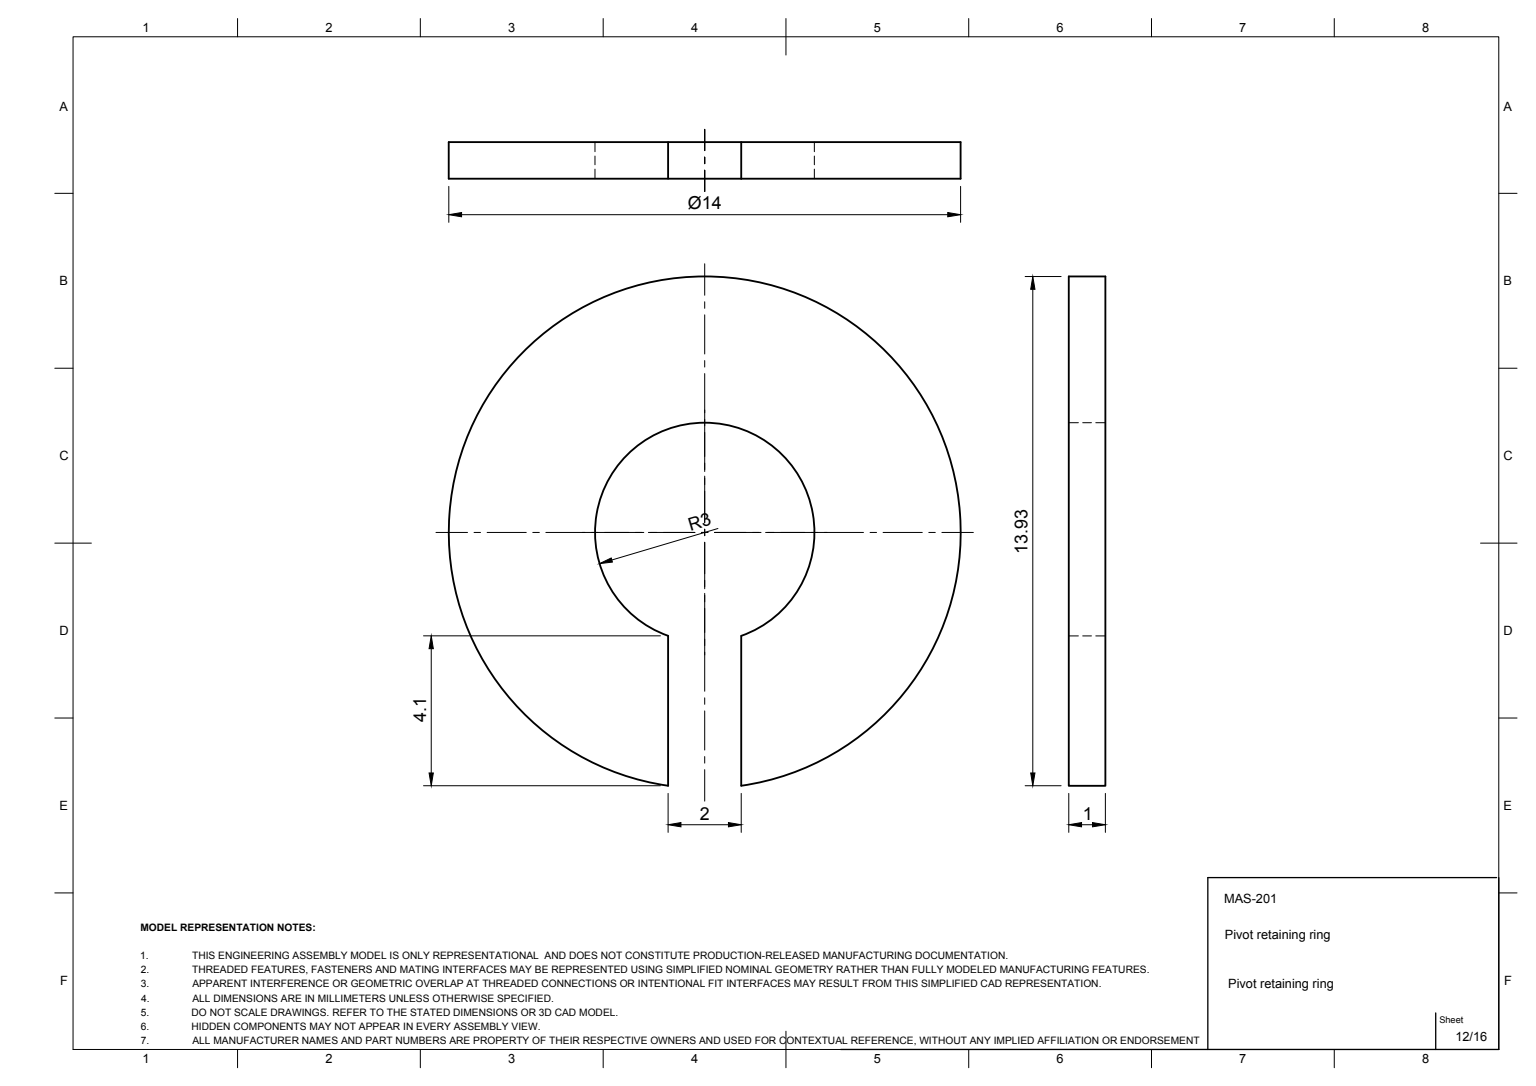
ISO-10303-21;
HEADER;
/* Generated by software containing ST-Developer
 * from STEP Tools, Inc. (www.steptools.com) 
 */

FILE_DESCRIPTION(
/* description */ ('Independent manual two-gate roller-track escapement for nominal30mm d
iameter20mm wide feed rollers. Opposed gates are driven by native capt
ured pin-slot loops with positive curved-slot travel stops at\X\B116de
g. Repeated gate/pin/washer/clip instances, adapted native common bear
ing families, full retaining lips and rotating polymer grip. External 
workpieces, gravity feeder/incline and mount anchors outside assembly.
 No powered-feed compatibility, impact, capacity, safety, force, wear 
or life rating.'),
/* implementation_level */ '2;1');

FILE_NAME(
/* name */ 'Pivot retaining ring.step',
/* time_stamp */ '2026-11-08T18:43:23-08:00',
/* author */ (''),
/* organization */ (''),
/* preprocessor_version */ 'ST-DEVELOPER v20.2',
/* originating_system */ 'Autodesk Translation Framework v15.17.0.0',
/* authorisation */ '');

FILE_SCHEMA (('AUTOMOTIVE_DESIGN { 1 0 10303 214 3 1 1 }'));
ENDSEC;

DATA;
#10=MECHANICAL_DESIGN_GEOMETRIC_PRESENTATION_REPRESENTATION('',(#466),#19863);
#428=SHAPE_REPRESENTATION_RELATIONSHIP('SRR','None',#19946,#447);
#447=ADVANCED_BREP_SHAPE_REPRESENTATION('',(#485),#19855);
#466=STYLED_ITEM('',(#20044),#485);
#485=MANIFOLD_SOLID_BREP('Body1',#6435);
#850=LINE('',#15919,#1315);
#851=LINE('',#15921,#1316);
#852=LINE('',#15923,#1317);
#853=LINE('',#15924,#1318);
#854=LINE('',#15928,#1319);
#855=LINE('',#15930,#1320);
#856=LINE('',#15932,#1321);
#857=LINE('',#15933,#1322);
#1315=VECTOR('',#8264,10.);
#1316=VECTOR('',#8265,10.);
#1317=VECTOR('',#8266,10.);
#1318=VECTOR('',#8267,10.);
#1319=VECTOR('',#8270,10.);
#1320=VECTOR('',#8271,10.);
#1321=VECTOR('',#8272,10.);
#1322=VECTOR('',#8273,10.);
#1554=CYLINDRICAL_SURFACE('',#7015,3.);
#1555=CYLINDRICAL_SURFACE('',#7017,7.);
#1937=FACE_OUTER_BOUND('',#2352,.T.);
#1938=FACE_OUTER_BOUND('',#2353,.T.);
#1939=FACE_OUTER_BOUND('',#2354,.T.);
#1940=FACE_OUTER_BOUND('',#2355,.T.);
#1941=FACE_OUTER_BOUND('',#2356,.T.);
#1942=FACE_OUTER_BOUND('',#2357,.T.);
#2352=EDGE_LOOP('',(#5409,#5410,#5411,#5412));
#2353=EDGE_LOOP('',(#5413,#5414,#5415,#5416));
#2354=EDGE_LOOP('',(#5417,#5418,#5419,#5420));
#2355=EDGE_LOOP('',(#5421,#5422,#5423,#5424));
#2356=EDGE_LOOP('',(#5425,#5426,#5427,#5428));
#2357=EDGE_LOOP('',(#5429,#5430,#5431,#5432));
#2574=CIRCLE('',#7013,7.);
#2575=CIRCLE('',#7014,3.);
#2576=CIRCLE('',#7016,3.);
#2577=CIRCLE('',#7018,7.);
#3048=VERTEX_POINT('',#15917);
#3049=VERTEX_POINT('',#15918);
#3050=VERTEX_POINT('',#15920);
#3051=VERTEX_POINT('',#15922);
#3052=VERTEX_POINT('',#15926);
#3053=VERTEX_POINT('',#15927);
#3054=VERTEX_POINT('',#15929);
#3055=VERTEX_POINT('',#15931);
#3863=EDGE_CURVE('',#3048,#3049,#850,.T.);
#3864=EDGE_CURVE('',#3050,#3048,#851,.T.);
#3865=EDGE_CURVE('',#3051,#3050,#852,.T.);
#3866=EDGE_CURVE('',#3049,#3051,#853,.T.);
#3867=EDGE_CURVE('',#3052,#3053,#854,.T.);
#3868=EDGE_CURVE('',#3054,#3052,#855,.T.);
#3869=EDGE_CURVE('',#3055,#3054,#856,.T.);
#3870=EDGE_CURVE('',#3053,#3055,#857,.T.);
#3871=EDGE_CURVE('',#3050,#3055,#2574,.T.);
#3872=EDGE_CURVE('',#3053,#3048,#2575,.T.);
#3873=EDGE_CURVE('',#3052,#3049,#2576,.T.);
#3874=EDGE_CURVE('',#3051,#3054,#2577,.T.);
#5409=ORIENTED_EDGE('',*,*,#3863,.F.);
#5410=ORIENTED_EDGE('',*,*,#3864,.F.);
#5411=ORIENTED_EDGE('',*,*,#3865,.F.);
#5412=ORIENTED_EDGE('',*,*,#3866,.F.);
#5413=ORIENTED_EDGE('',*,*,#3867,.F.);
#5414=ORIENTED_EDGE('',*,*,#3868,.F.);
#5415=ORIENTED_EDGE('',*,*,#3869,.F.);
#5416=ORIENTED_EDGE('',*,*,#3870,.F.);
#5417=ORIENTED_EDGE('',*,*,#3870,.T.);
#5418=ORIENTED_EDGE('',*,*,#3871,.F.);
#5419=ORIENTED_EDGE('',*,*,#3864,.T.);
#5420=ORIENTED_EDGE('',*,*,#3872,.F.);
#5421=ORIENTED_EDGE('',*,*,#3867,.T.);
#5422=ORIENTED_EDGE('',*,*,#3872,.T.);
#5423=ORIENTED_EDGE('',*,*,#3863,.T.);
#5424=ORIENTED_EDGE('',*,*,#3873,.F.);
#5425=ORIENTED_EDGE('',*,*,#3869,.T.);
#5426=ORIENTED_EDGE('',*,*,#3874,.F.);
#5427=ORIENTED_EDGE('',*,*,#3865,.T.);
#5428=ORIENTED_EDGE('',*,*,#3871,.T.);
#5429=ORIENTED_EDGE('',*,*,#3868,.T.);
#5430=ORIENTED_EDGE('',*,*,#3873,.T.);
#5431=ORIENTED_EDGE('',*,*,#3866,.T.);
#5432=ORIENTED_EDGE('',*,*,#3874,.T.);
#6026=PLANE('',#7010);
#6027=PLANE('',#7011);
#6028=PLANE('',#7012);
#6029=PLANE('',#7019);
#6316=ADVANCED_FACE('',(#1937),#6026,.F.);
#6317=ADVANCED_FACE('',(#1938),#6027,.F.);
#6318=ADVANCED_FACE('',(#1939),#6028,.F.);
#6319=ADVANCED_FACE('',(#1940),#1554,.F.);
#6320=ADVANCED_FACE('',(#1941),#1555,.T.);
#6321=ADVANCED_FACE('',(#1942),#6029,.T.);
#6435=CLOSED_SHELL('',(#6316,#6317,#6318,#6319,#6320,#6321));
#7009=AXIS2_PLACEMENT_3D('',#15915,#8260,#8261);
#7010=AXIS2_PLACEMENT_3D('',#15916,#8262,#8263);
#7011=AXIS2_PLACEMENT_3D('',#15925,#8268,#8269);
#7012=AXIS2_PLACEMENT_3D('',#15934,#8274,#8275);
#7013=AXIS2_PLACEMENT_3D('',#15935,#8276,#8277);
#7014=AXIS2_PLACEMENT_3D('',#15936,#8278,#8279);
#7015=AXIS2_PLACEMENT_3D('',#15937,#8280,#8281);
#7016=AXIS2_PLACEMENT_3D('',#15938,#8282,#8283);
#7017=AXIS2_PLACEMENT_3D('',#15939,#8284,#8285);
#7018=AXIS2_PLACEMENT_3D('',#15940,#8286,#8287);
#7019=AXIS2_PLACEMENT_3D('',#15941,#8288,#8289);
#8260=DIRECTION('axis',(0.,0.,1.));
#8261=DIRECTION('refdir',(1.,0.,0.));
#8262=DIRECTION('center_axis',(-1.,0.,0.));
#8263=DIRECTION('ref_axis',(0.,1.,0.));
#8264=DIRECTION('',(0.,0.,1.));
#8265=DIRECTION('',(0.,-1.,0.));
#8266=DIRECTION('',(0.,0.,-1.));
#8267=DIRECTION('',(0.,1.,0.));
#8268=DIRECTION('center_axis',(1.,0.,0.));
#8269=DIRECTION('ref_axis',(0.,-1.,0.));
#8270=DIRECTION('',(0.,0.,-1.));
#8271=DIRECTION('',(0.,-1.,0.));
#8272=DIRECTION('',(0.,0.,1.));
#8273=DIRECTION('',(0.,1.,0.));
#8274=DIRECTION('center_axis',(0.,0.,1.));
#8275=DIRECTION('ref_axis',(1.,0.,0.));
#8276=DIRECTION('center_axis',(0.,0.,1.));
#8277=DIRECTION('ref_axis',(1.,0.,0.));
#8278=DIRECTION('center_axis',(0.,0.,-1.));
#8279=DIRECTION('ref_axis',(1.,0.,0.));
#8280=DIRECTION('center_axis',(0.,0.,1.));
#8281=DIRECTION('ref_axis',(6.12323399573677E-17,-1.,0.));
#8282=DIRECTION('center_axis',(0.,0.,-1.));
#8283=DIRECTION('ref_axis',(1.,0.,0.));
#8284=DIRECTION('center_axis',(0.,0.,1.));
#8285=DIRECTION('ref_axis',(6.12323399573677E-17,-1.,0.));
#8286=DIRECTION('center_axis',(0.,0.,1.));
#8287=DIRECTION('ref_axis',(1.,0.,0.));
#8288=DIRECTION('center_axis',(0.,0.,1.));
#8289=DIRECTION('ref_axis',(1.,0.,0.));
#15915=CARTESIAN_POINT('',(0.,0.,0.));
#15916=CARTESIAN_POINT('Origin',(-1.,0.,1.));
#15917=CARTESIAN_POINT('',(-1.,2.82842712474619,0.));
#15918=CARTESIAN_POINT('',(-1.,2.82842712474619,1.));
#15919=CARTESIAN_POINT('',(-1.,2.82842712474619,0.));
#15920=CARTESIAN_POINT('',(-1.,6.92820323027551,0.));
#15921=CARTESIAN_POINT('',(-1.,0.,0.));
#15922=CARTESIAN_POINT('',(-1.,6.92820323027551,1.));
#15923=CARTESIAN_POINT('',(-1.,6.92820323027551,0.));
#15924=CARTESIAN_POINT('',(-1.,0.,1.));
#15925=CARTESIAN_POINT('Origin',(1.,14.,1.));
#15926=CARTESIAN_POINT('',(1.,2.82842712474619,1.));
#15927=CARTESIAN_POINT('',(1.,2.82842712474619,0.));
#15928=CARTESIAN_POINT('',(1.,2.82842712474619,0.));
#15929=CARTESIAN_POINT('',(1.,6.92820323027551,1.));
#15930=CARTESIAN_POINT('',(1.,7.,1.));
#15931=CARTESIAN_POINT('',(1.,6.92820323027551,0.));
#15932=CARTESIAN_POINT('',(1.,6.92820323027551,0.));
#15933=CARTESIAN_POINT('',(1.,7.,0.));
#15934=CARTESIAN_POINT('Origin',(0.,0.,0.));
#15935=CARTESIAN_POINT('Origin',(0.,0.,0.));
#15936=CARTESIAN_POINT('Origin',(0.,0.,0.));
#15937=CARTESIAN_POINT('Origin',(0.,0.,0.));
#15938=CARTESIAN_POINT('Origin',(0.,0.,1.));
#15939=CARTESIAN_POINT('Origin',(0.,0.,0.));
#15940=CARTESIAN_POINT('Origin',(0.,0.,1.));
#15941=CARTESIAN_POINT('Origin',(0.,0.,1.));
#19834=UNCERTAINTY_MEASURE_WITH_UNIT(LENGTH_MEASURE(0.01),#19864,
'DISTANCE_ACCURACY_VALUE',
'Maximum model space distance between geometric entities at asserted c
onnectivities');
#19842=UNCERTAINTY_MEASURE_WITH_UNIT(LENGTH_MEASURE(0.01),#19864,
'DISTANCE_ACCURACY_VALUE',
'Maximum model space distance between geometric entities at asserted c
onnectivities');
#19855=(
GEOMETRIC_REPRESENTATION_CONTEXT(3)
GLOBAL_UNCERTAINTY_ASSIGNED_CONTEXT((#19834))
GLOBAL_UNIT_ASSIGNED_CONTEXT((#19864,#19866,#19867))
REPRESENTATION_CONTEXT('','3D')
);
#19863=(
GEOMETRIC_REPRESENTATION_CONTEXT(3)
GLOBAL_UNCERTAINTY_ASSIGNED_CONTEXT((#19842))
GLOBAL_UNIT_ASSIGNED_CONTEXT((#19864,#19866,#19867))
REPRESENTATION_CONTEXT('','3D')
);
#19864=(
LENGTH_UNIT()
NAMED_UNIT(*)
SI_UNIT(.MILLI.,.METRE.)
);
#19866=(
NAMED_UNIT(*)
PLANE_ANGLE_UNIT()
SI_UNIT($,.RADIAN.)
);
#19867=(
NAMED_UNIT(*)
SI_UNIT($,.STERADIAN.)
SOLID_ANGLE_UNIT()
);
#19880=SHAPE_DEFINITION_REPRESENTATION(#19900,#19946);
#19900=PRODUCT_DEFINITION_SHAPE('',$,#19967);
#19946=SHAPE_REPRESENTATION('',(#7009),#19855);
#19954=PRODUCT_DEFINITION_CONTEXT('part definition',#20016,'design');
#19967=PRODUCT_DEFINITION('Pivot retaining ring','Pivot retaining ring',
#19987,#19954);
#19987=PRODUCT_DEFINITION_FORMATION('',$,#20030);
#20016=APPLICATION_CONTEXT(
'Core Data for Automotive Mechanical Design Process');
#20017=PRODUCT_CONTEXT('part definition',#20016,'mechanical');
#20030=PRODUCT('Pivot retaining ring','Pivot retaining ring',$,(#20017));
#20044=PRESENTATION_STYLE_ASSIGNMENT((#20051));
#20051=SURFACE_STYLE_USAGE(.BOTH.,#20058);
#20058=SURFACE_SIDE_STYLE('',(#20065));
#20065=SURFACE_STYLE_FILL_AREA(#20072);
#20072=FILL_AREA_STYLE('Dark gray',(#20079));
#20079=FILL_AREA_STYLE_COLOUR('Dark gray',#20086);
#20086=COLOUR_RGB('Dark gray',0.250980392156863,0.282352941176471,0.32156862745098);
ENDSEC;
END-ISO-10303-21;
